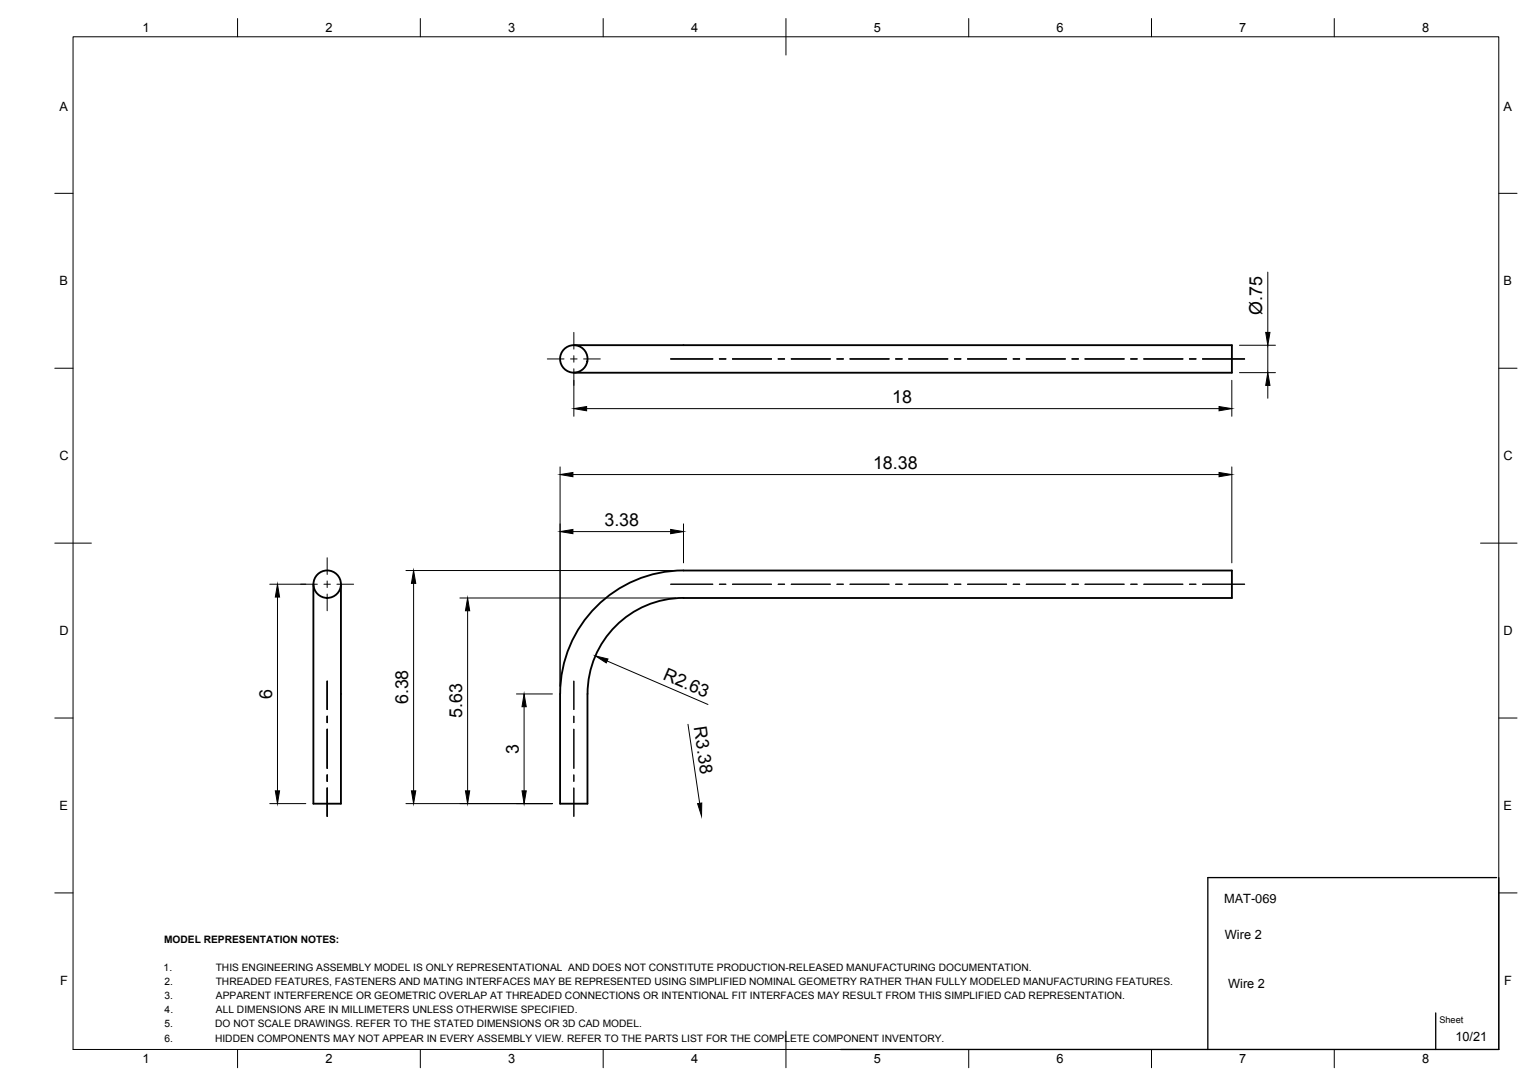
ISO-10303-21;
HEADER;
/* Generated by software containing ST-Developer
 * from STEP Tools, Inc. (www.steptools.com) 
 */

FILE_DESCRIPTION(
/* description */ ('CAx-IF Rec.Pracs.---Representation and Presentation of Product Manufa
cturing Information (PMI)---4.0---2014-10-13'),
/* implementation_level */ '2;1');

FILE_NAME(
/* name */ 'Wire 2.step',
/* time_stamp */ '2026-10-24T15:08:39-07:00',
/* author */ (''),
/* organization */ (''),
/* preprocessor_version */ 'ST-DEVELOPER v20.2',
/* originating_system */ 'Autodesk Translation Framework v15.17.0.0',
/* authorisation */ '');

FILE_SCHEMA (('AP242_MANAGED_MODEL_BASED_3D_ENGINEERING_MIM_LF { 1 0 10303 442 2 1 4 }'));
ENDSEC;

DATA;
#10=MECHANICAL_DESIGN_GEOMETRIC_PRESENTATION_REPRESENTATION('',(#827),#50081);
#774=TOROIDAL_SURFACE('',#10445,0.003,0.000375);
#787=SHAPE_REPRESENTATION_RELATIONSHIP('SRR','None',#50155,#807);
#807=ADVANCED_BREP_SHAPE_REPRESENTATION('',(#847),#50068);
#827=STYLED_ITEM('',(#50262),#847);
#847=MANIFOLD_SOLID_BREP('Body1',#9872);
#956=PLANE('',#10451);
#957=PLANE('',#10452);
#1266=FACE_OUTER_BOUND('',#1838,.T.);
#1267=FACE_OUTER_BOUND('',#1839,.T.);
#1268=FACE_OUTER_BOUND('',#1840,.T.);
#1269=FACE_OUTER_BOUND('',#1841,.T.);
#1270=FACE_OUTER_BOUND('',#1842,.T.);
#1838=EDGE_LOOP('',(#7016,#7017,#7018,#7019,#7020));
#1839=EDGE_LOOP('',(#7021,#7022,#7023,#7024,#7025,#7026));
#1840=EDGE_LOOP('',(#7027,#7028,#7029,#7030,#7031));
#1841=EDGE_LOOP('',(#7032));
#1842=EDGE_LOOP('',(#7033));
#2399=LINE('',#18102,#2977);
#2400=LINE('',#18114,#2978);
#2977=VECTOR('',#11865,0.000375);
#2978=VECTOR('',#11880,0.000375);
#3545=CIRCLE('',#10442,0.00037500000001);
#3546=CIRCLE('',#10443,0.00037500000001);
#3547=CIRCLE('',#10444,0.00037500000001);
#3548=CIRCLE('',#10446,0.002625);
#3549=CIRCLE('',#10447,0.00037500000001);
#3550=CIRCLE('',#10448,0.00037500000001);
#3551=CIRCLE('',#10450,0.00037500000001);
#4044=VERTEX_POINT('',#18099);
#4045=VERTEX_POINT('',#18101);
#4046=VERTEX_POINT('',#18103);
#4047=VERTEX_POINT('',#18107);
#4048=VERTEX_POINT('',#18109);
#4049=VERTEX_POINT('',#18113);
#5161=EDGE_CURVE('',#4044,#4044,#3545,.T.);
#5162=EDGE_CURVE('',#4044,#4045,#2399,.T.);
#5163=EDGE_CURVE('',#4045,#4046,#3546,.T.);
#5164=EDGE_CURVE('',#4046,#4045,#3547,.T.);
#5165=EDGE_CURVE('',#4046,#4047,#3548,.T.);
#5166=EDGE_CURVE('',#4047,#4048,#3549,.T.);
#5167=EDGE_CURVE('',#4048,#4047,#3550,.T.);
#5168=EDGE_CURVE('',#4048,#4049,#2400,.T.);
#5169=EDGE_CURVE('',#4049,#4049,#3551,.T.);
#7016=ORIENTED_EDGE('',*,*,#5161,.F.);
#7017=ORIENTED_EDGE('',*,*,#5162,.T.);
#7018=ORIENTED_EDGE('',*,*,#5163,.T.);
#7019=ORIENTED_EDGE('',*,*,#5164,.T.);
#7020=ORIENTED_EDGE('',*,*,#5162,.F.);
#7021=ORIENTED_EDGE('',*,*,#5164,.F.);
#7022=ORIENTED_EDGE('',*,*,#5165,.T.);
#7023=ORIENTED_EDGE('',*,*,#5166,.T.);
#7024=ORIENTED_EDGE('',*,*,#5167,.T.);
#7025=ORIENTED_EDGE('',*,*,#5165,.F.);
#7026=ORIENTED_EDGE('',*,*,#5163,.F.);
#7027=ORIENTED_EDGE('',*,*,#5167,.F.);
#7028=ORIENTED_EDGE('',*,*,#5168,.T.);
#7029=ORIENTED_EDGE('',*,*,#5169,.T.);
#7030=ORIENTED_EDGE('',*,*,#5168,.F.);
#7031=ORIENTED_EDGE('',*,*,#5166,.F.);
#7032=ORIENTED_EDGE('',*,*,#5161,.T.);
#7033=ORIENTED_EDGE('',*,*,#5169,.F.);
#9182=CYLINDRICAL_SURFACE('',#10441,0.000375);
#9183=CYLINDRICAL_SURFACE('',#10449,0.000375);
#9488=ADVANCED_FACE('',(#1266),#9182,.T.);
#9489=ADVANCED_FACE('',(#1267),#774,.T.);
#9490=ADVANCED_FACE('',(#1268),#9183,.T.);
#9491=ADVANCED_FACE('',(#1269),#956,.T.);
#9492=ADVANCED_FACE('',(#1270),#957,.F.);
#9872=CLOSED_SHELL('',(#9488,#9489,#9490,#9491,#9492));
#10440=AXIS2_PLACEMENT_3D('',#18097,#11859,#11860);
#10441=AXIS2_PLACEMENT_3D('',#18098,#11861,#11862);
#10442=AXIS2_PLACEMENT_3D('',#18100,#11863,#11864);
#10443=AXIS2_PLACEMENT_3D('',#18104,#11866,#11867);
#10444=AXIS2_PLACEMENT_3D('',#18105,#11868,#11869);
#10445=AXIS2_PLACEMENT_3D('',#18106,#11870,#11871);
#10446=AXIS2_PLACEMENT_3D('',#18108,#11872,#11873);
#10447=AXIS2_PLACEMENT_3D('',#18110,#11874,#11875);
#10448=AXIS2_PLACEMENT_3D('',#18111,#11876,#11877);
#10449=AXIS2_PLACEMENT_3D('',#18112,#11878,#11879);
#10450=AXIS2_PLACEMENT_3D('',#18115,#11881,#11882);
#10451=AXIS2_PLACEMENT_3D('',#18116,#11883,#11884);
#10452=AXIS2_PLACEMENT_3D('',#18117,#11885,#11886);
#11859=DIRECTION('axis',(0.,0.,1.));
#11860=DIRECTION('refdir',(1.,0.,0.));
#11861=DIRECTION('center_axis',(-6.74488507274914E-15,1.49880108324396E-15,
-1.));
#11862=DIRECTION('ref_axis',(-0.173648177666927,-0.984807753012209,-3.04793925546002E-16));
#11863=DIRECTION('center_axis',(2.62550741678841E-11,-4.62916846043658E-12,
-1.));
#11864=DIRECTION('ref_axis',(-0.173648177666927,-0.984807753012209,-3.04793925548737E-16));
#11865=DIRECTION('',(6.74488507274914E-15,-1.49880108324396E-15,1.));
#11866=DIRECTION('center_axis',(2.62550741678841E-11,-4.62916846043658E-12,
-1.));
#11867=DIRECTION('ref_axis',(-0.173648177666927,-0.984807753012209,-3.04793925548737E-16));
#11868=DIRECTION('center_axis',(2.62550741678841E-11,-4.62916846043658E-12,
-1.));
#11869=DIRECTION('ref_axis',(-0.173648177666927,-0.984807753012209,-3.04793925548737E-16));
#11870=DIRECTION('center_axis',(0.173648177666927,0.984807753012209,1.41609297436625E-15));
#11871=DIRECTION('ref_axis',(-6.16790569236198E-15,2.05596856412066E-15,
-1.));
#11872=DIRECTION('center_axis',(-0.173648177666927,-0.984807753012209,-1.41609297436625E-15));
#11873=DIRECTION('ref_axis',(-5.78605122952035E-15,2.45817543460173E-15,
-1.));
#11874=DIRECTION('center_axis',(0.984807753012209,-0.173648177666927,-6.9026791896102E-15));
#11875=DIRECTION('ref_axis',(-0.173648177666927,-0.984807753012209,-1.41609297436625E-15));
#11876=DIRECTION('center_axis',(0.984807753012209,-0.173648177666927,-6.9026791896102E-15));
#11877=DIRECTION('ref_axis',(-0.173648177666927,-0.984807753012209,-1.41609297436625E-15));
#11878=DIRECTION('center_axis',(0.984807753012209,-0.173648177666927,-6.9026791896102E-15));
#11879=DIRECTION('ref_axis',(-0.173648177666927,-0.984807753012209,-1.41609297436625E-15));
#11880=DIRECTION('',(-0.984807753012209,0.173648177666927,6.9026791896102E-15));
#11881=DIRECTION('center_axis',(0.984807753012209,-0.173648177666927,-6.9026791896102E-15));
#11882=DIRECTION('ref_axis',(-0.173648177666927,-0.984807753012209,-1.41609297436625E-15));
#11883=DIRECTION('center_axis',(-6.46591174117934E-15,1.44961055799008E-15,
-1.));
#11884=DIRECTION('ref_axis',(-0.173648177666927,-0.984807753012209,-3.04793925546006E-16));
#11885=DIRECTION('center_axis',(0.984807753012209,-0.173648177666927,-6.9026791896102E-15));
#11886=DIRECTION('ref_axis',(6.74488507274914E-15,-1.49880108324396E-15,
1.));
#18097=CARTESIAN_POINT('',(0.,0.,0.));
#18098=CARTESIAN_POINT('Origin',(-0.00676047226650036,-0.0387559860193906,
0.000824146758145397));
#18099=CARTESIAN_POINT('',(-0.00669535419987528,-0.038386683112011,-0.00217585328655808));
#18100=CARTESIAN_POINT('Origin',(-0.00676047226651023,-0.0387559860193889,
-0.00217585328654808));
#18101=CARTESIAN_POINT('',(-0.00669535419987526,-0.038386683112011,0.000824146758165397));
#18102=CARTESIAN_POINT('',(-0.00669535419987526,-0.038386683112011,0.000824146758145397));
#18103=CARTESIAN_POINT('',(-0.00712977517389963,-0.038690867952762,0.000824146758145399));
#18104=CARTESIAN_POINT('Origin',(-0.00676047226651021,-0.0387559860193889,
0.000824146758155397));
#18105=CARTESIAN_POINT('Origin',(-0.00676047226651021,-0.0387559860193889,
0.000824146758155397));
#18106=CARTESIAN_POINT('Origin',(-0.00971489552553699,-0.0382350414863898,
0.000824146758145418));
#18107=CARTESIAN_POINT('',(-0.00971489552554682,-0.0382350414863881,0.00344914675814542));
#18108=CARTESIAN_POINT('Origin',(-0.00971489552553699,-0.0382350414863898,
0.000824146758145418));
#18109=CARTESIAN_POINT('',(-0.0096497774589217,-0.0378657385790085,0.00382414675814542));
#18110=CARTESIAN_POINT('Origin',(-0.00971489552554682,-0.0382350414863881,
0.00382414675815542));
#18111=CARTESIAN_POINT('Origin',(-0.00971489552554682,-0.0382350414863881,
0.00382414675815542));
#18112=CARTESIAN_POINT('Origin',(-0.0244870118207201,-0.0356303188213859,
0.00382414675814552));
#18113=CARTESIAN_POINT('',(-0.0244218937541048,-0.0352610159140046,0.00382414675814552));
#18114=CARTESIAN_POINT('',(-0.024421893754095,-0.0352610159140063,0.00382414675814552));
#18115=CARTESIAN_POINT('Origin',(-0.0244870118207299,-0.0356303188213842,
0.00382414675815552));
#18116=CARTESIAN_POINT('Origin',(-0.00676047226650038,-0.0387559860193906,
-0.00217585328655808));
#18117=CARTESIAN_POINT('Origin',(-0.0244870118207201,-0.0356303188213859,
0.00382414675814552));
#50046=UNCERTAINTY_MEASURE_WITH_UNIT(LENGTH_MEASURE(1.E-5),#50082,
'DISTANCE_ACCURACY_VALUE',
'Maximum model space distance between geometric entities at asserted c
onnectivities');
#50059=UNCERTAINTY_MEASURE_WITH_UNIT(LENGTH_MEASURE(1.E-5),#50082,
'DISTANCE_ACCURACY_VALUE',
'Maximum model space distance between geometric entities at asserted c
onnectivities');
#50068=(
GEOMETRIC_REPRESENTATION_CONTEXT(3)
GLOBAL_UNCERTAINTY_ASSIGNED_CONTEXT((#50046))
GLOBAL_UNIT_ASSIGNED_CONTEXT((#50082,#50083,#50084))
REPRESENTATION_CONTEXT('','3D')
);
#50081=(
GEOMETRIC_REPRESENTATION_CONTEXT(3)
GLOBAL_UNCERTAINTY_ASSIGNED_CONTEXT((#50059))
GLOBAL_UNIT_ASSIGNED_CONTEXT((#50082,#50083,#50084))
REPRESENTATION_CONTEXT('','3D')
);
#50082=(
LENGTH_UNIT()
NAMED_UNIT(*)
SI_UNIT($,.METRE.)
);
#50083=(
NAMED_UNIT(*)
PLANE_ANGLE_UNIT()
SI_UNIT($,.RADIAN.)
);
#50084=(
NAMED_UNIT(*)
SI_UNIT($,.STERADIAN.)
SOLID_ANGLE_UNIT()
);
#50093=SHAPE_DEFINITION_REPRESENTATION(#50114,#50155);
#50114=PRODUCT_DEFINITION_SHAPE('',$,#50177);
#50155=SHAPE_REPRESENTATION('',(#10440),#50068);
#50168=PRODUCT_DEFINITION_CONTEXT('part definition',#50233,'design');
#50177=PRODUCT_DEFINITION('Wire 2','Wire 2',#50198,#50168);
#50198=PRODUCT_DEFINITION_FORMATION('',$,#50243);
#50233=APPLICATION_CONTEXT('Managed model based 3d engineering');
#50234=PRODUCT_CONTEXT('part definition',#50233,'mechanical');
#50243=PRODUCT('Wire 2','Wire 2','Wire',(#50234));
#50262=PRESENTATION_STYLE_ASSIGNMENT((#50269));
#50269=SURFACE_STYLE_USAGE(.BOTH.,#50276);
#50276=SURFACE_SIDE_STYLE('',(#50283));
#50283=SURFACE_STYLE_FILL_AREA(#50290);
#50290=FILL_AREA_STYLE('Opaque(48,59,150)',(#50297));
#50297=FILL_AREA_STYLE_COLOUR('Opaque(48,59,150)',#50304);
#50304=COLOUR_RGB('Opaque(48,59,150)',0.188235294117647,0.231372549019608,
0.588235294117647);
ENDSEC;
END-ISO-10303-21;
